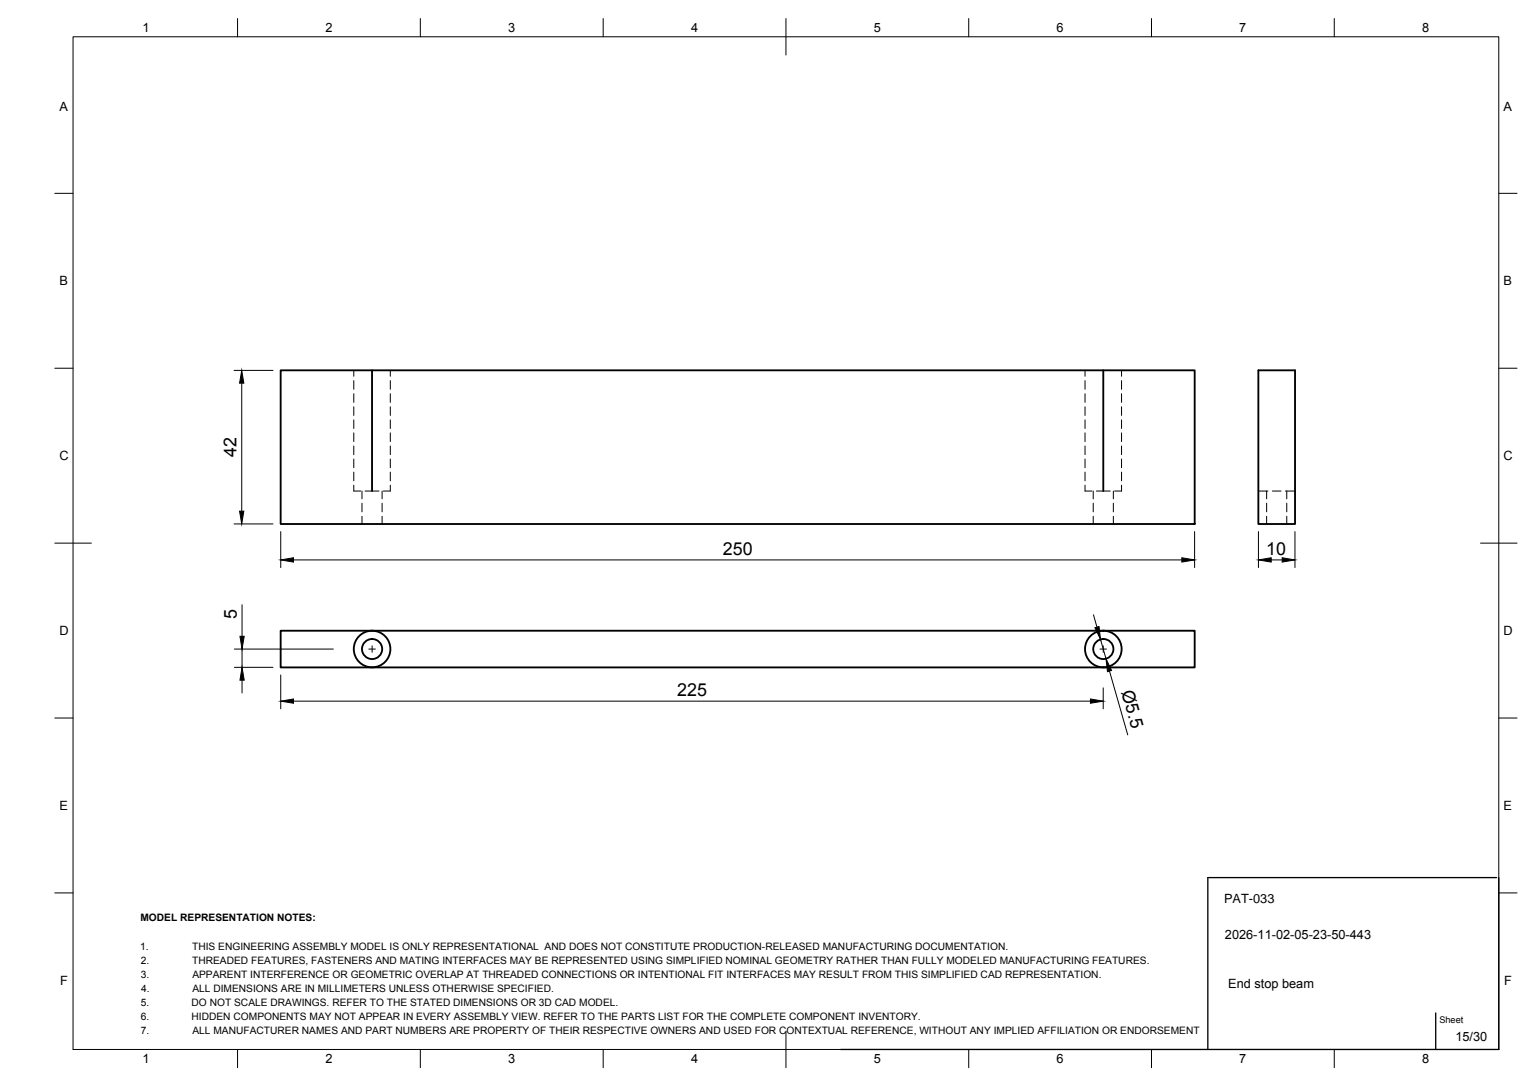
ISO-10303-21;
HEADER;
/* Generated by software containing ST-Developer
 * from STEP Tools, Inc. (www.steptools.com) 
 */

FILE_DESCRIPTION(
/* description */ ('Dual-rail gantry carriage'),
/* implementation_level */ '2;1');

FILE_NAME(
/* name */ 'End stop beam.step',
/* time_stamp */ '2026-10-27T10:49:15-07:00',
/* author */ (''),
/* organization */ (''),
/* preprocessor_version */ 'ST-DEVELOPER v20.2',
/* originating_system */ 'Autodesk Translation Framework v15.17.0.0',
/* authorisation */ '');

FILE_SCHEMA (('AUTOMOTIVE_DESIGN { 1 0 10303 214 3 1 1 }'));
ENDSEC;

DATA;
#10=MECHANICAL_DESIGN_GEOMETRIC_PRESENTATION_REPRESENTATION('',(#595),#12804);
#533=SHAPE_REPRESENTATION_RELATIONSHIP('SRR','None',#13011,#564);
#564=ADVANCED_BREP_SHAPE_REPRESENTATION('',(#626),#12781);
#595=STYLED_ITEM('',(#13233),#626);
#626=MANIFOLD_SOLID_BREP('Body1',#7373);
#682=FACE_BOUND('',#1560,.T.);
#683=FACE_BOUND('',#1564,.T.);
#684=FACE_BOUND('',#1575,.T.);
#685=FACE_BOUND('',#1576,.T.);
#824=PLANE('',#7880);
#825=PLANE('',#7888);
#826=PLANE('',#7890);
#827=PLANE('',#7891);
#828=PLANE('',#7892);
#829=PLANE('',#7897);
#830=PLANE('',#7898);
#831=PLANE('',#7899);
#832=PLANE('',#7900);
#833=PLANE('',#7901);
#1128=FACE_OUTER_BOUND('',#1557,.T.);
#1129=FACE_OUTER_BOUND('',#1558,.T.);
#1130=FACE_OUTER_BOUND('',#1559,.T.);
#1131=FACE_OUTER_BOUND('',#1561,.T.);
#1132=FACE_OUTER_BOUND('',#1562,.T.);
#1133=FACE_OUTER_BOUND('',#1563,.T.);
#1134=FACE_OUTER_BOUND('',#1565,.T.);
#1135=FACE_OUTER_BOUND('',#1566,.T.);
#1136=FACE_OUTER_BOUND('',#1567,.T.);
#1137=FACE_OUTER_BOUND('',#1568,.T.);
#1138=FACE_OUTER_BOUND('',#1569,.T.);
#1139=FACE_OUTER_BOUND('',#1570,.T.);
#1140=FACE_OUTER_BOUND('',#1571,.T.);
#1141=FACE_OUTER_BOUND('',#1572,.T.);
#1142=FACE_OUTER_BOUND('',#1573,.T.);
#1143=FACE_OUTER_BOUND('',#1574,.T.);
#1557=EDGE_LOOP('',(#5427,#5428,#5429,#5430));
#1558=EDGE_LOOP('',(#5431,#5432,#5433,#5434));
#1559=EDGE_LOOP('',(#5435,#5436));
#1560=EDGE_LOOP('',(#5437));
#1561=EDGE_LOOP('',(#5438,#5439,#5440,#5441));
#1562=EDGE_LOOP('',(#5442,#5443,#5444,#5445));
#1563=EDGE_LOOP('',(#5446,#5447));
#1564=EDGE_LOOP('',(#5448));
#1565=EDGE_LOOP('',(#5449,#5450,#5451,#5452));
#1566=EDGE_LOOP('',(#5453,#5454,#5455,#5456));
#1567=EDGE_LOOP('',(#5457,#5458,#5459,#5460));
#1568=EDGE_LOOP('',(#5461,#5462,#5463,#5464));
#1569=EDGE_LOOP('',(#5465,#5466,#5467,#5468));
#1570=EDGE_LOOP('',(#5469,#5470,#5471,#5472));
#1571=EDGE_LOOP('',(#5473,#5474,#5475,#5476,#5477,#5478,#5479,#5480,#5481,
#5482));
#1572=EDGE_LOOP('',(#5483,#5484,#5485,#5486));
#1573=EDGE_LOOP('',(#5487,#5488,#5489,#5490,#5491,#5492,#5493,#5494,#5495,
#5496));
#1574=EDGE_LOOP('',(#5497,#5498,#5499,#5500));
#1575=EDGE_LOOP('',(#5501));
#1576=EDGE_LOOP('',(#5502));
#2088=LINE('',#11084,#2797);
#2089=LINE('',#11088,#2798);
#2090=LINE('',#11091,#2799);
#2091=LINE('',#11093,#2800);
#2092=LINE('',#11101,#2801);
#2093=LINE('',#11105,#2802);
#2094=LINE('',#11108,#2803);
#2095=LINE('',#11110,#2804);
#2096=LINE('',#11117,#2805);
#2097=LINE('',#11119,#2806);
#2098=LINE('',#11120,#2807);
#2099=LINE('',#11122,#2808);
#2100=LINE('',#11123,#2809);
#2101=LINE('',#11126,#2810);
#2102=LINE('',#11128,#2811);
#2103=LINE('',#11129,#2812);
#2104=LINE('',#11133,#2813);
#2105=LINE('',#11137,#2814);
#2106=LINE('',#11141,#2815);
#2107=LINE('',#11142,#2816);
#2108=LINE('',#11143,#2817);
#2109=LINE('',#11146,#2818);
#2110=LINE('',#11147,#2819);
#2111=LINE('',#11150,#2820);
#2112=LINE('',#11151,#2821);
#2113=LINE('',#11153,#2822);
#2797=VECTOR('',#8895,1.);
#2798=VECTOR('',#8898,1.);
#2799=VECTOR('',#8903,1.);
#2800=VECTOR('',#8906,1.);
#2801=VECTOR('',#8915,1.);
#2802=VECTOR('',#8918,1.);
#2803=VECTOR('',#8923,1.);
#2804=VECTOR('',#8926,1.);
#2805=VECTOR('',#8935,1.);
#2806=VECTOR('',#8936,1.);
#2807=VECTOR('',#8937,1.);
#2808=VECTOR('',#8940,1.);
#2809=VECTOR('',#8941,1.);
#2810=VECTOR('',#8944,1.);
#2811=VECTOR('',#8945,1.);
#2812=VECTOR('',#8946,1.);
#2813=VECTOR('',#8951,0.275);
#2814=VECTOR('',#8956,0.275);
#2815=VECTOR('',#8959,1.);
#2816=VECTOR('',#8960,1.);
#2817=VECTOR('',#8961,1.);
#2818=VECTOR('',#8964,1.);
#2819=VECTOR('',#8965,1.);
#2820=VECTOR('',#8968,1.);
#2821=VECTOR('',#8969,1.);
#2822=VECTOR('',#8972,1.);
#3406=CIRCLE('',#7875,0.5);
#3407=CIRCLE('',#7876,0.5);
#3408=CIRCLE('',#7878,0.5);
#3409=CIRCLE('',#7879,0.5);
#3410=CIRCLE('',#7881,0.275);
#3411=CIRCLE('',#7883,0.5);
#3412=CIRCLE('',#7884,0.5);
#3413=CIRCLE('',#7886,0.5);
#3414=CIRCLE('',#7887,0.5);
#3415=CIRCLE('',#7889,0.275);
#3416=CIRCLE('',#7894,0.275);
#3417=CIRCLE('',#7896,0.275);
#3686=VERTEX_POINT('',#11082);
#3687=VERTEX_POINT('',#11083);
#3688=VERTEX_POINT('',#11085);
#3689=VERTEX_POINT('',#11087);
#3690=VERTEX_POINT('',#11096);
#3691=VERTEX_POINT('',#11099);
#3692=VERTEX_POINT('',#11100);
#3693=VERTEX_POINT('',#11102);
#3694=VERTEX_POINT('',#11104);
#3695=VERTEX_POINT('',#11113);
#3696=VERTEX_POINT('',#11116);
#3697=VERTEX_POINT('',#11118);
#3698=VERTEX_POINT('',#11125);
#3699=VERTEX_POINT('',#11127);
#3700=VERTEX_POINT('',#11131);
#3701=VERTEX_POINT('',#11135);
#3702=VERTEX_POINT('',#11139);
#3703=VERTEX_POINT('',#11140);
#3704=VERTEX_POINT('',#11145);
#3705=VERTEX_POINT('',#11149);
#4336=EDGE_CURVE('',#3686,#3687,#2088,.T.);
#4337=EDGE_CURVE('',#3688,#3687,#3406,.T.);
#4338=EDGE_CURVE('',#3689,#3688,#2089,.T.);
#4339=EDGE_CURVE('',#3686,#3689,#3407,.T.);
#4340=EDGE_CURVE('',#3686,#3687,#2090,.T.);
#4341=EDGE_CURVE('',#3689,#3686,#3408,.T.);
#4342=EDGE_CURVE('',#3689,#3688,#2091,.T.);
#4343=EDGE_CURVE('',#3687,#3688,#3409,.T.);
#4344=EDGE_CURVE('',#3690,#3690,#3410,.T.);
#4345=EDGE_CURVE('',#3691,#3692,#2092,.T.);
#4346=EDGE_CURVE('',#3693,#3692,#3411,.T.);
#4347=EDGE_CURVE('',#3694,#3693,#2093,.T.);
#4348=EDGE_CURVE('',#3691,#3694,#3412,.T.);
#4349=EDGE_CURVE('',#3691,#3692,#2094,.T.);
#4350=EDGE_CURVE('',#3694,#3691,#3413,.T.);
#4351=EDGE_CURVE('',#3694,#3693,#2095,.T.);
#4352=EDGE_CURVE('',#3692,#3693,#3414,.T.);
#4353=EDGE_CURVE('',#3695,#3695,#3415,.T.);
#4354=EDGE_CURVE('',#3692,#3696,#2096,.T.);
#4355=EDGE_CURVE('',#3696,#3697,#2097,.T.);
#4356=EDGE_CURVE('',#3697,#3693,#2098,.T.);
#4357=EDGE_CURVE('',#3687,#3692,#2099,.T.);
#4358=EDGE_CURVE('',#3693,#3688,#2100,.T.);
#4359=EDGE_CURVE('',#3688,#3698,#2101,.T.);
#4360=EDGE_CURVE('',#3698,#3699,#2102,.T.);
#4361=EDGE_CURVE('',#3699,#3687,#2103,.T.);
#4362=EDGE_CURVE('',#3700,#3700,#3416,.T.);
#4363=EDGE_CURVE('',#3700,#3690,#2104,.T.);
#4364=EDGE_CURVE('',#3701,#3701,#3417,.T.);
#4365=EDGE_CURVE('',#3701,#3695,#2105,.T.);
#4366=EDGE_CURVE('',#3702,#3703,#2106,.T.);
#4367=EDGE_CURVE('',#3703,#3697,#2107,.T.);
#4368=EDGE_CURVE('',#3702,#3696,#2108,.T.);
#4369=EDGE_CURVE('',#3704,#3702,#2109,.T.);
#4370=EDGE_CURVE('',#3704,#3699,#2110,.T.);
#4371=EDGE_CURVE('',#3705,#3704,#2111,.T.);
#4372=EDGE_CURVE('',#3705,#3698,#2112,.T.);
#4373=EDGE_CURVE('',#3703,#3705,#2113,.T.);
#5427=ORIENTED_EDGE('',*,*,#4336,.T.);
#5428=ORIENTED_EDGE('',*,*,#4337,.F.);
#5429=ORIENTED_EDGE('',*,*,#4338,.F.);
#5430=ORIENTED_EDGE('',*,*,#4339,.F.);
#5431=ORIENTED_EDGE('',*,*,#4340,.F.);
#5432=ORIENTED_EDGE('',*,*,#4341,.F.);
#5433=ORIENTED_EDGE('',*,*,#4342,.T.);
#5434=ORIENTED_EDGE('',*,*,#4343,.F.);
#5435=ORIENTED_EDGE('',*,*,#4341,.T.);
#5436=ORIENTED_EDGE('',*,*,#4339,.T.);
#5437=ORIENTED_EDGE('',*,*,#4344,.F.);
#5438=ORIENTED_EDGE('',*,*,#4345,.T.);
#5439=ORIENTED_EDGE('',*,*,#4346,.F.);
#5440=ORIENTED_EDGE('',*,*,#4347,.F.);
#5441=ORIENTED_EDGE('',*,*,#4348,.F.);
#5442=ORIENTED_EDGE('',*,*,#4349,.F.);
#5443=ORIENTED_EDGE('',*,*,#4350,.F.);
#5444=ORIENTED_EDGE('',*,*,#4351,.T.);
#5445=ORIENTED_EDGE('',*,*,#4352,.F.);
#5446=ORIENTED_EDGE('',*,*,#4350,.T.);
#5447=ORIENTED_EDGE('',*,*,#4348,.T.);
#5448=ORIENTED_EDGE('',*,*,#4353,.F.);
#5449=ORIENTED_EDGE('',*,*,#4346,.T.);
#5450=ORIENTED_EDGE('',*,*,#4354,.T.);
#5451=ORIENTED_EDGE('',*,*,#4355,.T.);
#5452=ORIENTED_EDGE('',*,*,#4356,.T.);
#5453=ORIENTED_EDGE('',*,*,#4337,.T.);
#5454=ORIENTED_EDGE('',*,*,#4357,.T.);
#5455=ORIENTED_EDGE('',*,*,#4352,.T.);
#5456=ORIENTED_EDGE('',*,*,#4358,.T.);
#5457=ORIENTED_EDGE('',*,*,#4343,.T.);
#5458=ORIENTED_EDGE('',*,*,#4359,.T.);
#5459=ORIENTED_EDGE('',*,*,#4360,.T.);
#5460=ORIENTED_EDGE('',*,*,#4361,.T.);
#5461=ORIENTED_EDGE('',*,*,#4362,.F.);
#5462=ORIENTED_EDGE('',*,*,#4363,.T.);
#5463=ORIENTED_EDGE('',*,*,#4344,.T.);
#5464=ORIENTED_EDGE('',*,*,#4363,.F.);
#5465=ORIENTED_EDGE('',*,*,#4364,.F.);
#5466=ORIENTED_EDGE('',*,*,#4365,.T.);
#5467=ORIENTED_EDGE('',*,*,#4353,.T.);
#5468=ORIENTED_EDGE('',*,*,#4365,.F.);
#5469=ORIENTED_EDGE('',*,*,#4366,.T.);
#5470=ORIENTED_EDGE('',*,*,#4367,.T.);
#5471=ORIENTED_EDGE('',*,*,#4355,.F.);
#5472=ORIENTED_EDGE('',*,*,#4368,.F.);
#5473=ORIENTED_EDGE('',*,*,#4369,.T.);
#5474=ORIENTED_EDGE('',*,*,#4368,.T.);
#5475=ORIENTED_EDGE('',*,*,#4354,.F.);
#5476=ORIENTED_EDGE('',*,*,#4345,.F.);
#5477=ORIENTED_EDGE('',*,*,#4349,.T.);
#5478=ORIENTED_EDGE('',*,*,#4357,.F.);
#5479=ORIENTED_EDGE('',*,*,#4336,.F.);
#5480=ORIENTED_EDGE('',*,*,#4340,.T.);
#5481=ORIENTED_EDGE('',*,*,#4361,.F.);
#5482=ORIENTED_EDGE('',*,*,#4370,.F.);
#5483=ORIENTED_EDGE('',*,*,#4371,.T.);
#5484=ORIENTED_EDGE('',*,*,#4370,.T.);
#5485=ORIENTED_EDGE('',*,*,#4360,.F.);
#5486=ORIENTED_EDGE('',*,*,#4372,.F.);
#5487=ORIENTED_EDGE('',*,*,#4373,.T.);
#5488=ORIENTED_EDGE('',*,*,#4372,.T.);
#5489=ORIENTED_EDGE('',*,*,#4359,.F.);
#5490=ORIENTED_EDGE('',*,*,#4342,.F.);
#5491=ORIENTED_EDGE('',*,*,#4338,.T.);
#5492=ORIENTED_EDGE('',*,*,#4358,.F.);
#5493=ORIENTED_EDGE('',*,*,#4351,.F.);
#5494=ORIENTED_EDGE('',*,*,#4347,.T.);
#5495=ORIENTED_EDGE('',*,*,#4356,.F.);
#5496=ORIENTED_EDGE('',*,*,#4367,.F.);
#5497=ORIENTED_EDGE('',*,*,#4373,.F.);
#5498=ORIENTED_EDGE('',*,*,#4366,.F.);
#5499=ORIENTED_EDGE('',*,*,#4369,.F.);
#5500=ORIENTED_EDGE('',*,*,#4371,.F.);
#5501=ORIENTED_EDGE('',*,*,#4362,.T.);
#5502=ORIENTED_EDGE('',*,*,#4364,.T.);
#6909=CYLINDRICAL_SURFACE('',#7874,0.5);
#6910=CYLINDRICAL_SURFACE('',#7877,0.5);
#6911=CYLINDRICAL_SURFACE('',#7882,0.5);
#6912=CYLINDRICAL_SURFACE('',#7885,0.5);
#6913=CYLINDRICAL_SURFACE('',#7893,0.275);
#6914=CYLINDRICAL_SURFACE('',#7895,0.275);
#7054=ADVANCED_FACE('',(#1128),#6909,.F.);
#7055=ADVANCED_FACE('',(#1129),#6910,.F.);
#7056=ADVANCED_FACE('',(#1130,#682),#824,.T.);
#7057=ADVANCED_FACE('',(#1131),#6911,.F.);
#7058=ADVANCED_FACE('',(#1132),#6912,.F.);
#7059=ADVANCED_FACE('',(#1133,#683),#825,.T.);
#7060=ADVANCED_FACE('',(#1134),#826,.T.);
#7061=ADVANCED_FACE('',(#1135),#827,.T.);
#7062=ADVANCED_FACE('',(#1136),#828,.T.);
#7063=ADVANCED_FACE('',(#1137),#6913,.F.);
#7064=ADVANCED_FACE('',(#1138),#6914,.F.);
#7065=ADVANCED_FACE('',(#1139),#829,.T.);
#7066=ADVANCED_FACE('',(#1140),#830,.T.);
#7067=ADVANCED_FACE('',(#1141),#831,.T.);
#7068=ADVANCED_FACE('',(#1142),#832,.T.);
#7069=ADVANCED_FACE('',(#1143,#684,#685),#833,.F.);
#7373=CLOSED_SHELL('',(#7054,#7055,#7056,#7057,#7058,#7059,#7060,#7061,
#7062,#7063,#7064,#7065,#7066,#7067,#7068,#7069));
#7873=AXIS2_PLACEMENT_3D('',#11080,#8891,#8892);
#7874=AXIS2_PLACEMENT_3D('',#11081,#8893,#8894);
#7875=AXIS2_PLACEMENT_3D('',#11086,#8896,#8897);
#7876=AXIS2_PLACEMENT_3D('',#11089,#8899,#8900);
#7877=AXIS2_PLACEMENT_3D('',#11090,#8901,#8902);
#7878=AXIS2_PLACEMENT_3D('',#11092,#8904,#8905);
#7879=AXIS2_PLACEMENT_3D('',#11094,#8907,#8908);
#7880=AXIS2_PLACEMENT_3D('',#11095,#8909,#8910);
#7881=AXIS2_PLACEMENT_3D('',#11097,#8911,#8912);
#7882=AXIS2_PLACEMENT_3D('',#11098,#8913,#8914);
#7883=AXIS2_PLACEMENT_3D('',#11103,#8916,#8917);
#7884=AXIS2_PLACEMENT_3D('',#11106,#8919,#8920);
#7885=AXIS2_PLACEMENT_3D('',#11107,#8921,#8922);
#7886=AXIS2_PLACEMENT_3D('',#11109,#8924,#8925);
#7887=AXIS2_PLACEMENT_3D('',#11111,#8927,#8928);
#7888=AXIS2_PLACEMENT_3D('',#11112,#8929,#8930);
#7889=AXIS2_PLACEMENT_3D('',#11114,#8931,#8932);
#7890=AXIS2_PLACEMENT_3D('',#11115,#8933,#8934);
#7891=AXIS2_PLACEMENT_3D('',#11121,#8938,#8939);
#7892=AXIS2_PLACEMENT_3D('',#11124,#8942,#8943);
#7893=AXIS2_PLACEMENT_3D('',#11130,#8947,#8948);
#7894=AXIS2_PLACEMENT_3D('',#11132,#8949,#8950);
#7895=AXIS2_PLACEMENT_3D('',#11134,#8952,#8953);
#7896=AXIS2_PLACEMENT_3D('',#11136,#8954,#8955);
#7897=AXIS2_PLACEMENT_3D('',#11138,#8957,#8958);
#7898=AXIS2_PLACEMENT_3D('',#11144,#8962,#8963);
#7899=AXIS2_PLACEMENT_3D('',#11148,#8966,#8967);
#7900=AXIS2_PLACEMENT_3D('',#11152,#8970,#8971);
#7901=AXIS2_PLACEMENT_3D('',#11154,#8973,#8974);
#8891=DIRECTION('axis',(0.,0.,1.));
#8892=DIRECTION('refdir',(1.,0.,0.));
#8893=DIRECTION('center_axis',(0.,0.,1.));
#8894=DIRECTION('ref_axis',(1.,0.,0.));
#8895=DIRECTION('',(0.,0.,1.));
#8896=DIRECTION('center_axis',(0.,0.,-1.));
#8897=DIRECTION('ref_axis',(1.,0.,0.));
#8898=DIRECTION('',(0.,0.,1.));
#8899=DIRECTION('center_axis',(0.,0.,1.));
#8900=DIRECTION('ref_axis',(1.,0.,0.));
#8901=DIRECTION('center_axis',(0.,0.,1.));
#8902=DIRECTION('ref_axis',(1.,0.,0.));
#8903=DIRECTION('',(0.,0.,1.));
#8904=DIRECTION('center_axis',(0.,0.,1.));
#8905=DIRECTION('ref_axis',(1.,0.,0.));
#8906=DIRECTION('',(0.,0.,1.));
#8907=DIRECTION('center_axis',(0.,0.,-1.));
#8908=DIRECTION('ref_axis',(1.,0.,0.));
#8909=DIRECTION('center_axis',(0.,0.,1.));
#8910=DIRECTION('ref_axis',(1.,0.,0.));
#8911=DIRECTION('center_axis',(0.,0.,1.));
#8912=DIRECTION('ref_axis',(1.,0.,0.));
#8913=DIRECTION('center_axis',(0.,0.,1.));
#8914=DIRECTION('ref_axis',(1.,0.,0.));
#8915=DIRECTION('',(0.,0.,1.));
#8916=DIRECTION('center_axis',(0.,0.,-1.));
#8917=DIRECTION('ref_axis',(1.,0.,0.));
#8918=DIRECTION('',(0.,0.,1.));
#8919=DIRECTION('center_axis',(0.,0.,1.));
#8920=DIRECTION('ref_axis',(1.,0.,0.));
#8921=DIRECTION('center_axis',(0.,0.,1.));
#8922=DIRECTION('ref_axis',(1.,0.,0.));
#8923=DIRECTION('',(0.,0.,1.));
#8924=DIRECTION('center_axis',(0.,0.,1.));
#8925=DIRECTION('ref_axis',(1.,0.,0.));
#8926=DIRECTION('',(0.,0.,1.));
#8927=DIRECTION('center_axis',(0.,0.,-1.));
#8928=DIRECTION('ref_axis',(1.,0.,0.));
#8929=DIRECTION('center_axis',(0.,0.,1.));
#8930=DIRECTION('ref_axis',(1.,0.,0.));
#8931=DIRECTION('center_axis',(0.,0.,1.));
#8932=DIRECTION('ref_axis',(1.,0.,0.));
#8933=DIRECTION('center_axis',(0.,0.,1.));
#8934=DIRECTION('ref_axis',(1.,0.,0.));
#8935=DIRECTION('',(0.,1.,0.));
#8936=DIRECTION('',(-1.,0.,0.));
#8937=DIRECTION('',(0.,-1.,0.));
#8938=DIRECTION('center_axis',(0.,0.,1.));
#8939=DIRECTION('ref_axis',(1.,0.,0.));
#8940=DIRECTION('',(0.,1.,0.));
#8941=DIRECTION('',(0.,-1.,0.));
#8942=DIRECTION('center_axis',(0.,0.,1.));
#8943=DIRECTION('ref_axis',(1.,0.,0.));
#8944=DIRECTION('',(0.,-1.,0.));
#8945=DIRECTION('',(1.,0.,0.));
#8946=DIRECTION('',(0.,1.,0.));
#8947=DIRECTION('center_axis',(0.,0.,1.));
#8948=DIRECTION('ref_axis',(1.,0.,0.));
#8949=DIRECTION('center_axis',(0.,0.,1.));
#8950=DIRECTION('ref_axis',(1.,0.,0.));
#8951=DIRECTION('',(0.,0.,1.));
#8952=DIRECTION('center_axis',(0.,0.,1.));
#8953=DIRECTION('ref_axis',(1.,0.,0.));
#8954=DIRECTION('center_axis',(0.,0.,1.));
#8955=DIRECTION('ref_axis',(1.,0.,0.));
#8956=DIRECTION('',(0.,0.,1.));
#8957=DIRECTION('center_axis',(0.,1.,0.));
#8958=DIRECTION('ref_axis',(-1.,0.,0.));
#8959=DIRECTION('',(-1.,0.,0.));
#8960=DIRECTION('',(0.,0.,1.));
#8961=DIRECTION('',(0.,0.,1.));
#8962=DIRECTION('center_axis',(1.,0.,0.));
#8963=DIRECTION('ref_axis',(0.,1.,0.));
#8964=DIRECTION('',(0.,1.,0.));
#8965=DIRECTION('',(0.,0.,1.));
#8966=DIRECTION('center_axis',(0.,-1.,0.));
#8967=DIRECTION('ref_axis',(1.,0.,0.));
#8968=DIRECTION('',(1.,0.,0.));
#8969=DIRECTION('',(0.,0.,1.));
#8970=DIRECTION('center_axis',(-1.,0.,0.));
#8971=DIRECTION('ref_axis',(0.,-1.,0.));
#8972=DIRECTION('',(0.,-1.,0.));
#8973=DIRECTION('center_axis',(0.,0.,1.));
#8974=DIRECTION('ref_axis',(1.,0.,0.));
#11080=CARTESIAN_POINT('',(0.,0.,0.));
#11081=CARTESIAN_POINT('Origin',(7.5,-10.,2.9));
#11082=CARTESIAN_POINT('',(8.,-10.,2.9));
#11083=CARTESIAN_POINT('',(8.,-10.,6.2));
#11084=CARTESIAN_POINT('',(8.,-10.,2.9));
#11085=CARTESIAN_POINT('',(7.,-10.,6.2));
#11086=CARTESIAN_POINT('Origin',(7.5,-10.,6.2));
#11087=CARTESIAN_POINT('',(7.,-10.,2.9));
#11088=CARTESIAN_POINT('',(7.,-10.,2.9));
#11089=CARTESIAN_POINT('Origin',(7.5,-10.,2.9));
#11090=CARTESIAN_POINT('Origin',(7.5,-10.,2.9));
#11091=CARTESIAN_POINT('',(8.,-10.,2.9));
#11092=CARTESIAN_POINT('Origin',(7.5,-10.,2.9));
#11093=CARTESIAN_POINT('',(7.,-10.,2.9));
#11094=CARTESIAN_POINT('Origin',(7.5,-10.,6.2));
#11095=CARTESIAN_POINT('Origin',(7.5,-10.,2.9));
#11096=CARTESIAN_POINT('',(7.225,-10.,2.9));
#11097=CARTESIAN_POINT('Origin',(7.5,-10.,2.9));
#11098=CARTESIAN_POINT('Origin',(7.5,10.,2.9));
#11099=CARTESIAN_POINT('',(8.,10.,2.9));
#11100=CARTESIAN_POINT('',(8.,10.,6.2));
#11101=CARTESIAN_POINT('',(8.,10.,2.9));
#11102=CARTESIAN_POINT('',(7.,10.,6.2));
#11103=CARTESIAN_POINT('Origin',(7.5,10.,6.2));
#11104=CARTESIAN_POINT('',(7.,10.,2.9));
#11105=CARTESIAN_POINT('',(7.,10.,2.9));
#11106=CARTESIAN_POINT('Origin',(7.5,10.,2.9));
#11107=CARTESIAN_POINT('Origin',(7.5,10.,2.9));
#11108=CARTESIAN_POINT('',(8.,10.,2.9));
#11109=CARTESIAN_POINT('Origin',(7.5,10.,2.9));
#11110=CARTESIAN_POINT('',(7.,10.,2.9));
#11111=CARTESIAN_POINT('Origin',(7.5,10.,6.2));
#11112=CARTESIAN_POINT('Origin',(7.5,10.,2.9));
#11113=CARTESIAN_POINT('',(7.225,10.,2.9));
#11114=CARTESIAN_POINT('Origin',(7.5,10.,2.9));
#11115=CARTESIAN_POINT('Origin',(7.5,0.,6.2));
#11116=CARTESIAN_POINT('',(8.,12.5,6.2));
#11117=CARTESIAN_POINT('',(8.,-12.5,6.2));
#11118=CARTESIAN_POINT('',(7.,12.5,6.2));
#11119=CARTESIAN_POINT('',(8.,12.5,6.2));
#11120=CARTESIAN_POINT('',(7.,12.5,6.2));
#11121=CARTESIAN_POINT('Origin',(7.5,0.,6.2));
#11122=CARTESIAN_POINT('',(8.,-12.5,6.2));
#11123=CARTESIAN_POINT('',(7.,12.5,6.2));
#11124=CARTESIAN_POINT('Origin',(7.5,0.,6.2));
#11125=CARTESIAN_POINT('',(7.,-12.5,6.2));
#11126=CARTESIAN_POINT('',(7.,12.5,6.2));
#11127=CARTESIAN_POINT('',(8.,-12.5,6.2));
#11128=CARTESIAN_POINT('',(7.,-12.5,6.2));
#11129=CARTESIAN_POINT('',(8.,-12.5,6.2));
#11130=CARTESIAN_POINT('Origin',(7.5,-10.,1.9));
#11131=CARTESIAN_POINT('',(7.225,-10.,2.));
#11132=CARTESIAN_POINT('Origin',(7.5,-10.,2.));
#11133=CARTESIAN_POINT('',(7.225,-10.,1.9));
#11134=CARTESIAN_POINT('Origin',(7.5,10.,1.9));
#11135=CARTESIAN_POINT('',(7.225,10.,2.));
#11136=CARTESIAN_POINT('Origin',(7.5,10.,2.));
#11137=CARTESIAN_POINT('',(7.225,10.,1.9));
#11138=CARTESIAN_POINT('Origin',(8.,12.5,2.));
#11139=CARTESIAN_POINT('',(8.,12.5,2.));
#11140=CARTESIAN_POINT('',(7.,12.5,2.));
#11141=CARTESIAN_POINT('',(8.,12.5,2.));
#11142=CARTESIAN_POINT('',(7.,12.5,2.));
#11143=CARTESIAN_POINT('',(8.,12.5,2.));
#11144=CARTESIAN_POINT('Origin',(8.,-12.5,2.));
#11145=CARTESIAN_POINT('',(8.,-12.5,2.));
#11146=CARTESIAN_POINT('',(8.,-12.5,2.));
#11147=CARTESIAN_POINT('',(8.,-12.5,2.));
#11148=CARTESIAN_POINT('Origin',(7.,-12.5,2.));
#11149=CARTESIAN_POINT('',(7.,-12.5,2.));
#11150=CARTESIAN_POINT('',(7.,-12.5,2.));
#11151=CARTESIAN_POINT('',(7.,-12.5,2.));
#11152=CARTESIAN_POINT('Origin',(7.,12.5,2.));
#11153=CARTESIAN_POINT('',(7.,12.5,2.));
#11154=CARTESIAN_POINT('Origin',(7.5,0.,2.));
#12745=UNCERTAINTY_MEASURE_WITH_UNIT(LENGTH_MEASURE(0.001),#12805,
'DISTANCE_ACCURACY_VALUE',
'Maximum model space distance between geometric entities at asserted c
onnectivities');
#12768=UNCERTAINTY_MEASURE_WITH_UNIT(LENGTH_MEASURE(0.001),#12805,
'DISTANCE_ACCURACY_VALUE',
'Maximum model space distance between geometric entities at asserted c
onnectivities');
#12781=(
GEOMETRIC_REPRESENTATION_CONTEXT(3)
GLOBAL_UNCERTAINTY_ASSIGNED_CONTEXT((#12745))
GLOBAL_UNIT_ASSIGNED_CONTEXT((#12805,#12807,#12808))
REPRESENTATION_CONTEXT('','3D')
);
#12804=(
GEOMETRIC_REPRESENTATION_CONTEXT(3)
GLOBAL_UNCERTAINTY_ASSIGNED_CONTEXT((#12768))
GLOBAL_UNIT_ASSIGNED_CONTEXT((#12805,#12807,#12808))
REPRESENTATION_CONTEXT('','3D')
);
#12805=(
LENGTH_UNIT()
NAMED_UNIT(*)
SI_UNIT(.CENTI.,.METRE.)
);
#12807=(
NAMED_UNIT(*)
PLANE_ANGLE_UNIT()
SI_UNIT($,.RADIAN.)
);
#12808=(
NAMED_UNIT(*)
SI_UNIT($,.STERADIAN.)
SOLID_ANGLE_UNIT()
);
#12821=SHAPE_DEFINITION_REPRESENTATION(#12856,#13011);
#12856=PRODUCT_DEFINITION_SHAPE('',$,#13047);
#13011=SHAPE_REPRESENTATION('',(#7873),#12781);
#13034=PRODUCT_DEFINITION_CONTEXT('part definition',#13141,'design');
#13047=PRODUCT_DEFINITION('End stop beam','End stop beam',#13082,#13034);
#13082=PRODUCT_DEFINITION_FORMATION('',$,#13155);
#13141=APPLICATION_CONTEXT(
'Core Data for Automotive Mechanical Design Process');
#13142=PRODUCT_CONTEXT('part definition',#13141,'mechanical');
#13155=PRODUCT('End stop beam','End stop beam','End stop beam',(#13142));
#13227=COLOUR_RGB('Light Blue',0.38,0.62,0.78);
#13228=FILL_AREA_STYLE_COLOUR('',#13227);
#13229=FILL_AREA_STYLE('',(#13228));
#13230=SURFACE_STYLE_FILL_AREA(#13229);
#13231=SURFACE_SIDE_STYLE('',(#13230));
#13232=SURFACE_STYLE_USAGE(.BOTH.,#13231);
#13233=PRESENTATION_STYLE_ASSIGNMENT((#13232));
ENDSEC;
END-ISO-10303-21;
